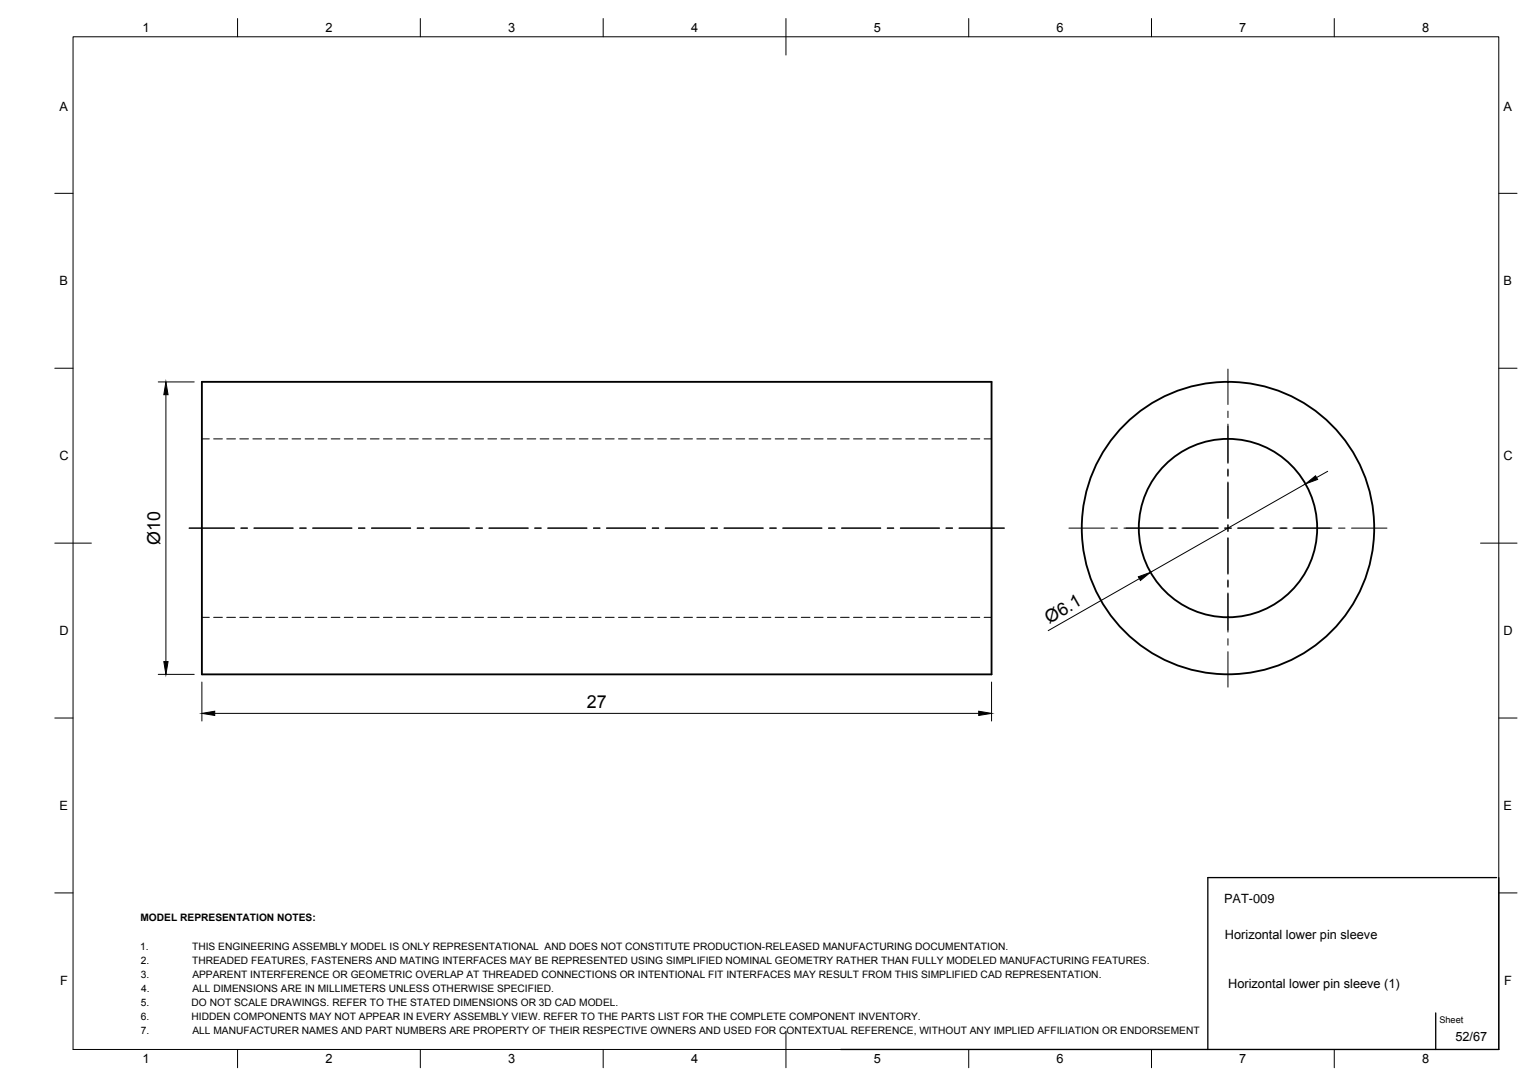
ISO-10303-21;
HEADER;
/* Generated by software containing ST-Developer
 * from STEP Tools, Inc. (www.steptools.com) 
 */

FILE_DESCRIPTION(
/* description */ ('Bell-crank linkage with push rods'),
/* implementation_level */ '2;1');

FILE_NAME(
/* name */ 'Horizontal lower pin sleeve (1).step',
/* time_stamp */ '2026-10-28T03:25:15-07:00',
/* author */ (''),
/* organization */ (''),
/* preprocessor_version */ 'ST-DEVELOPER v20.2',
/* originating_system */ 'Autodesk Translation Framework v15.17.0.0',
/* authorisation */ '');

FILE_SCHEMA (('AUTOMOTIVE_DESIGN { 1 0 10303 214 3 1 1 }'));
ENDSEC;

DATA;
#10=MECHANICAL_DESIGN_GEOMETRIC_PRESENTATION_REPRESENTATION('',(#653),#16678);
#537=SHAPE_REPRESENTATION_RELATIONSHIP('SRR','None',#16958,#591);
#591=ADVANCED_BREP_SHAPE_REPRESENTATION('',(#713),#16663);
#653=STYLED_ITEM('',(#17291),#713);
#713=MANIFOLD_SOLID_BREP('Body1',#8845);
#908=FACE_BOUND('',#2368,.T.);
#909=FACE_BOUND('',#2370,.T.);
#1183=PLANE('',#10330);
#1184=PLANE('',#10331);
#1660=FACE_OUTER_BOUND('',#2365,.T.);
#1661=FACE_OUTER_BOUND('',#2366,.T.);
#1662=FACE_OUTER_BOUND('',#2367,.T.);
#1663=FACE_OUTER_BOUND('',#2369,.T.);
#2365=EDGE_LOOP('',(#7647,#7648,#7649,#7650));
#2366=EDGE_LOOP('',(#7651,#7652,#7653,#7654));
#2367=EDGE_LOOP('',(#7655));
#2368=EDGE_LOOP('',(#7656));
#2369=EDGE_LOOP('',(#7657));
#2370=EDGE_LOOP('',(#7658));
#2964=LINE('',#15993,#3513);
#2965=LINE('',#15999,#3514);
#3513=VECTOR('',#12806,0.305);
#3514=VECTOR('',#12813,0.5);
#4027=CIRCLE('',#10325,0.305);
#4028=CIRCLE('',#10326,0.305);
#4029=CIRCLE('',#10328,0.5);
#4030=CIRCLE('',#10329,0.5);
#4694=VERTEX_POINT('',#15990);
#4695=VERTEX_POINT('',#15992);
#4696=VERTEX_POINT('',#15996);
#4697=VERTEX_POINT('',#15998);
#5701=EDGE_CURVE('',#4694,#4694,#4027,.T.);
#5702=EDGE_CURVE('',#4694,#4695,#2964,.T.);
#5703=EDGE_CURVE('',#4695,#4695,#4028,.T.);
#5704=EDGE_CURVE('',#4696,#4696,#4029,.T.);
#5705=EDGE_CURVE('',#4696,#4697,#2965,.T.);
#5706=EDGE_CURVE('',#4697,#4697,#4030,.T.);
#7647=ORIENTED_EDGE('',*,*,#5701,.F.);
#7648=ORIENTED_EDGE('',*,*,#5702,.T.);
#7649=ORIENTED_EDGE('',*,*,#5703,.T.);
#7650=ORIENTED_EDGE('',*,*,#5702,.F.);
#7651=ORIENTED_EDGE('',*,*,#5704,.F.);
#7652=ORIENTED_EDGE('',*,*,#5705,.T.);
#7653=ORIENTED_EDGE('',*,*,#5706,.T.);
#7654=ORIENTED_EDGE('',*,*,#5705,.F.);
#7655=ORIENTED_EDGE('',*,*,#5704,.T.);
#7656=ORIENTED_EDGE('',*,*,#5701,.T.);
#7657=ORIENTED_EDGE('',*,*,#5706,.F.);
#7658=ORIENTED_EDGE('',*,*,#5703,.F.);
#8230=CYLINDRICAL_SURFACE('',#10324,0.305);
#8231=CYLINDRICAL_SURFACE('',#10327,0.5);
#8685=ADVANCED_FACE('',(#1660),#8230,.F.);
#8686=ADVANCED_FACE('',(#1661),#8231,.T.);
#8687=ADVANCED_FACE('',(#1662,#908),#1183,.T.);
#8688=ADVANCED_FACE('',(#1663,#909),#1184,.F.);
#8845=CLOSED_SHELL('',(#8685,#8686,#8687,#8688));
#10323=AXIS2_PLACEMENT_3D('',#15988,#12800,#12801);
#10324=AXIS2_PLACEMENT_3D('',#15989,#12802,#12803);
#10325=AXIS2_PLACEMENT_3D('',#15991,#12804,#12805);
#10326=AXIS2_PLACEMENT_3D('',#15994,#12807,#12808);
#10327=AXIS2_PLACEMENT_3D('',#15995,#12809,#12810);
#10328=AXIS2_PLACEMENT_3D('',#15997,#12811,#12812);
#10329=AXIS2_PLACEMENT_3D('',#16000,#12814,#12815);
#10330=AXIS2_PLACEMENT_3D('',#16001,#12816,#12817);
#10331=AXIS2_PLACEMENT_3D('',#16002,#12818,#12819);
#12800=DIRECTION('axis',(0.,0.,1.));
#12801=DIRECTION('refdir',(1.,0.,0.));
#12802=DIRECTION('center_axis',(0.,0.,1.));
#12803=DIRECTION('ref_axis',(1.,0.,0.));
#12804=DIRECTION('center_axis',(0.,0.,-1.));
#12805=DIRECTION('ref_axis',(1.,0.,0.));
#12806=DIRECTION('',(0.,0.,-1.));
#12807=DIRECTION('center_axis',(0.,0.,-1.));
#12808=DIRECTION('ref_axis',(1.,0.,0.));
#12809=DIRECTION('center_axis',(0.,0.,1.));
#12810=DIRECTION('ref_axis',(1.,0.,0.));
#12811=DIRECTION('center_axis',(0.,0.,1.));
#12812=DIRECTION('ref_axis',(1.,0.,0.));
#12813=DIRECTION('',(0.,0.,-1.));
#12814=DIRECTION('center_axis',(0.,0.,1.));
#12815=DIRECTION('ref_axis',(1.,0.,0.));
#12816=DIRECTION('center_axis',(0.,0.,1.));
#12817=DIRECTION('ref_axis',(1.,0.,0.));
#12818=DIRECTION('center_axis',(0.,0.,1.));
#12819=DIRECTION('ref_axis',(1.,0.,0.));
#15988=CARTESIAN_POINT('',(0.,0.,0.));
#15989=CARTESIAN_POINT('Origin',(10.,2.,6.1));
#15990=CARTESIAN_POINT('',(9.695,2.,8.8));
#15991=CARTESIAN_POINT('Origin',(10.,2.,8.8));
#15992=CARTESIAN_POINT('',(9.695,2.,6.1));
#15993=CARTESIAN_POINT('',(9.695,2.,6.1));
#15994=CARTESIAN_POINT('Origin',(10.,2.,6.1));
#15995=CARTESIAN_POINT('Origin',(10.,2.,6.1));
#15996=CARTESIAN_POINT('',(9.5,2.,8.8));
#15997=CARTESIAN_POINT('Origin',(10.,2.,8.8));
#15998=CARTESIAN_POINT('',(9.5,2.,6.1));
#15999=CARTESIAN_POINT('',(9.5,2.,6.1));
#16000=CARTESIAN_POINT('Origin',(10.,2.,6.1));
#16001=CARTESIAN_POINT('Origin',(10.,2.,8.8));
#16002=CARTESIAN_POINT('Origin',(10.,2.,6.1));
#16599=UNCERTAINTY_MEASURE_WITH_UNIT(LENGTH_MEASURE(0.001),#16679,
'DISTANCE_ACCURACY_VALUE',
'Maximum model space distance between geometric entities at asserted c
onnectivities');
#16614=UNCERTAINTY_MEASURE_WITH_UNIT(LENGTH_MEASURE(0.001),#16679,
'DISTANCE_ACCURACY_VALUE',
'Maximum model space distance between geometric entities at asserted c
onnectivities');
#16663=(
GEOMETRIC_REPRESENTATION_CONTEXT(3)
GLOBAL_UNCERTAINTY_ASSIGNED_CONTEXT((#16599))
GLOBAL_UNIT_ASSIGNED_CONTEXT((#16679,#16681,#16682))
REPRESENTATION_CONTEXT('','3D')
);
#16678=(
GEOMETRIC_REPRESENTATION_CONTEXT(3)
GLOBAL_UNCERTAINTY_ASSIGNED_CONTEXT((#16614))
GLOBAL_UNIT_ASSIGNED_CONTEXT((#16679,#16681,#16682))
REPRESENTATION_CONTEXT('','3D')
);
#16679=(
LENGTH_UNIT()
NAMED_UNIT(*)
SI_UNIT(.CENTI.,.METRE.)
);
#16681=(
NAMED_UNIT(*)
PLANE_ANGLE_UNIT()
SI_UNIT($,.RADIAN.)
);
#16682=(
NAMED_UNIT(*)
SI_UNIT($,.STERADIAN.)
SOLID_ANGLE_UNIT()
);
#16731=SHAPE_DEFINITION_REPRESENTATION(#16805,#16958);
#16805=PRODUCT_DEFINITION_SHAPE('',$,#17022);
#16958=SHAPE_REPRESENTATION('',(#10323),#16663);
#16973=PRODUCT_DEFINITION_CONTEXT('part definition',#17164,'design');
#17022=PRODUCT_DEFINITION('Horizontal lower pin sleeve (1)',
'Horizontal lower pin sleeve (1)',#17085,#16973);
#17085=PRODUCT_DEFINITION_FORMATION('',$,#17214);
#17164=APPLICATION_CONTEXT(
'Core Data for Automotive Mechanical Design Process');
#17165=PRODUCT_CONTEXT('part definition',#17164,'mechanical');
#17214=PRODUCT('Horizontal lower pin sleeve (1)',
'Horizontal lower pin sleeve (1)','Horizontal lower pin sleeve (1)',(#17165));
#17285=COLOUR_RGB('Grey',0.48,0.52,0.57);
#17286=FILL_AREA_STYLE_COLOUR('',#17285);
#17287=FILL_AREA_STYLE('',(#17286));
#17288=SURFACE_STYLE_FILL_AREA(#17287);
#17289=SURFACE_SIDE_STYLE('',(#17288));
#17290=SURFACE_STYLE_USAGE(.BOTH.,#17289);
#17291=PRESENTATION_STYLE_ASSIGNMENT((#17290));
ENDSEC;
END-ISO-10303-21;
